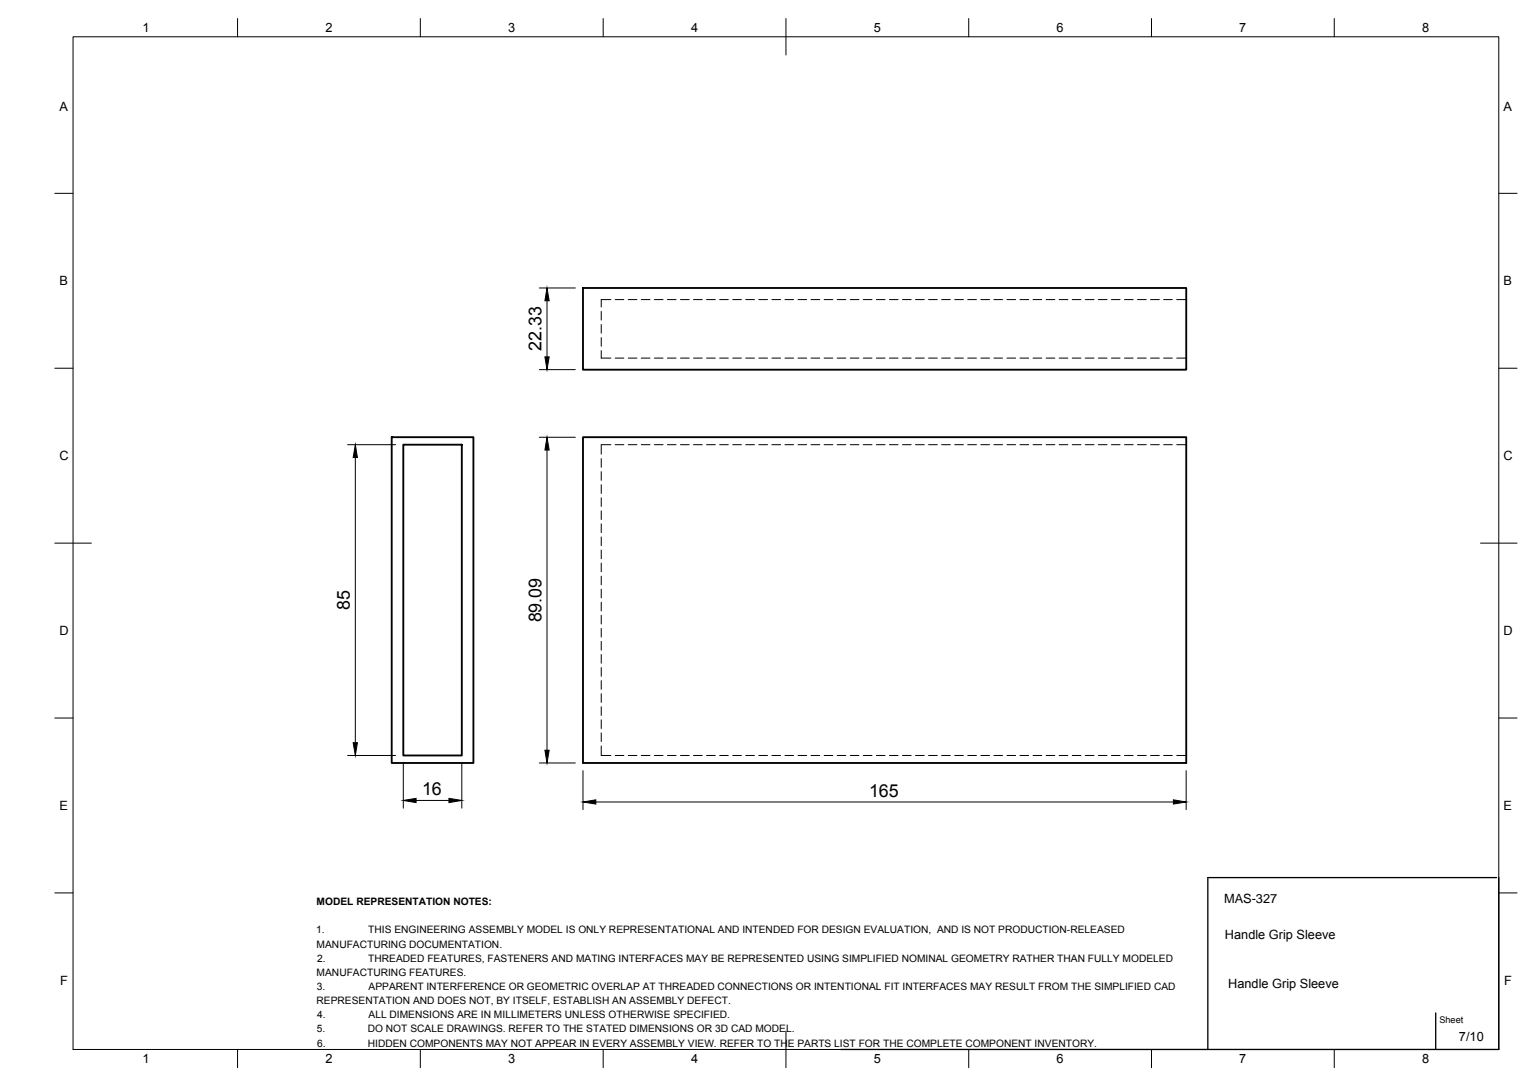
ISO-10303-21;
HEADER;
FILE_DESCRIPTION (('STEP AP214'),
    '1' );
FILE_NAME ('Handle Grip Sleeve.step',
    '2026-10-06T22:16:42',
    ( '' ),
    ( '' ),
    'SwSTEP 2.0',
    'SolidWorks 2025',
    '' );
FILE_SCHEMA (( 'AUTOMOTIVE_DESIGN' ));
ENDSEC;

DATA;
#37=ORIENTED_EDGE ( 'NONE', *, *, #161, .T. ) ;
#47=CARTESIAN_POINT ( 'NONE',  ( 2.004595370269653287, 635.3380690778678854, -0.8325491102011938205 ) ) ;
#122=CARTESIAN_POINT ( 'NONE',  ( -55.11860757350579831, 784.8075632535900468, -19.99999999999997868 ) ) ;
#123=ORIENTED_EDGE ( 'NONE', *, *, #17302, .F. ) ;
#161=EDGE_CURVE ( 'NONE', #6406, #8778, #2868, .T. ) ;
#223=ORIENTED_EDGE ( 'NONE', *, *, #18510, .T. ) ;
#234=PLANE ( 'NONE',  #15635 ) ;
#305=EDGE_CURVE ( 'NONE', #10554, #5083, #3643, .T. ) ;
#371=CARTESIAN_POINT ( 'NONE',  ( 0.08333186253070556937, 634.6318465664363657, -3.999999999999996447 ) ) ;
#441=DIRECTION ( 'NONE',  ( 0.000000000000000000, 0.000000000000000000, -1.000000000000000000 ) ) ;
#454=DIRECTION ( 'NONE',  ( 0.3450121214752279175, -0.9385982292947087080, 0.000000000000000000 ) ) ;
#567=CARTESIAN_POINT ( 'NONE',  ( -81.61981105773979550, 604.5992151483073940, -0.8325491102011938205 ) ) ;
#631=ORIENTED_EDGE ( 'NONE', *, *, #10728, .F. ) ;
#770=AXIS2_PLACEMENT_3D ( 'NONE', #10420, #3801, #12272 ) ;
#955=CARTESIAN_POINT ( 'NONE',  ( -134.9004869860375777, 755.4811543468929358, -19.99999999999996092 ) ) ;
#1022=CARTESIAN_POINT ( 'NONE',  ( -55.11860757350579831, 784.8075632535900468, -3.999999999999996447 ) ) ;
#1068=FACE_OUTER_BOUND ( 'NONE', #16645, .T. ) ;
#1109=ORIENTED_EDGE ( 'NONE', *, *, #17157, .T. ) ;
#1197=LINE ( 'NONE', #6263, #13695 ) ;
#1300=CARTESIAN_POINT ( 'NONE',  ( 0.08333186253067781379, 634.6318465664365931, -19.99999999999997868 ) ) ;
#1431=LINE ( 'NONE', #10574, #2685 ) ;
#1557=DIRECTION ( 'NONE',  ( -0.3450121214752279175, 0.9385982292947087080, 0.000000000000000000 ) ) ;
#1616=DIRECTION ( 'NONE',  ( 0.000000000000000000, 0.000000000000000000, -1.000000000000000000 ) ) ;
#1663=VECTOR ( 'NONE', #13216, 1000.000000000000114 ) ;
#1715=CARTESIAN_POINT ( 'NONE',  ( 0.08333186253067781379, 634.6318465664365931, -3.999999999999996447 ) ) ;
#1787=DIRECTION ( 'NONE',  ( 0.3450121214752279175, -0.9385982292947087080, -0.000000000000000000 ) ) ;
#1831=ORIENTED_EDGE ( 'NONE', *, *, #17120, .T. ) ;
#2049=ORIENTED_EDGE ( 'NONE', *, *, #6385, .T. ) ;
#2195=VECTOR ( 'NONE', #5994, 1000.000000000000000 ) ;
#2240=UNCERTAINTY_MEASURE_WITH_UNIT (LENGTH_MEASURE( 1.000000000000000082E-05 ), #9375, 'distance_accuracy_value', 'NONE');
#2256=ORIENTED_EDGE ( 'NONE', *, *, #305, .F. ) ;
#2403=CARTESIAN_POINT ( 'NONE',  ( 0.000000000000000000, 0.000000000000000000, 0.000000000000000000 ) ) ;
#2452=DIRECTION ( 'NONE',  ( 1.000000000000000000, 0.000000000000000000, -1.723963091245776585E-16 ) ) ;
#2568=LINE ( 'NONE', #2671, #12905 ) ;
#2635=FILL_AREA_STYLE ('',( #6156 ) ) ;
#2671=CARTESIAN_POINT ( 'NONE',  ( -138.5468111011521160, 759.4679229819337252, -0.8325491102011938205 ) ) ;
#2685=VECTOR ( 'NONE', #15626, 1000.000000000000000 ) ;
#2721=AXIS2_PLACEMENT_3D ( 'NONE', #1022, #14760, #2452 ) ;
#2868=LINE ( 'NONE', #18073, #21489 ) ;
#2903=ADVANCED_FACE ( 'NONE', ( #8379 ), #20176, .T. ) ;
#2927=VERTEX_POINT ( 'NONE', #11262 ) ;
#2952=VECTOR ( 'NONE', #1787, 1000.000000000000114 ) ;
#2972=AXIS2_PLACEMENT_3D ( 'NONE', #5225, #5530, #11012 ) ;
#3024=LINE ( 'NONE', #18003, #3512 ) ;
#3044=DIRECTION ( 'NONE',  ( -1.915514545828640705E-16, -7.041092946335507105E-17, -1.000000000000000000 ) ) ;
#3074=CARTESIAN_POINT ( 'NONE',  ( -81.61981105773979550, 604.5992151483073940, -23.16745088979876499 ) ) ;
#3090=ORIENTED_EDGE ( 'NONE', *, *, #18510, .F. ) ;
#3128=ORIENTED_EDGE ( 'NONE', *, *, #7265, .F. ) ;
#3197=LINE ( 'NONE', #6738, #17161 ) ;
#3211=FACE_OUTER_BOUND ( 'NONE', #21508, .T. ) ;
#3289=ORIENTED_EDGE ( 'NONE', *, *, #9467, .T. ) ;
#3512=VECTOR ( 'NONE', #12725, 1000.000000000000000 ) ;
#3514=ORIENTED_EDGE ( 'NONE', *, *, #12179, .F. ) ;
#3565=LINE ( 'NONE', #567, #6404 ) ;
#3643=LINE ( 'NONE', #5186, #7066 ) ;
#3693=FACE_OUTER_BOUND ( 'NONE', #13506, .T. ) ;
#3778=CARTESIAN_POINT ( 'NONE',  ( -55.11860757350579831, 784.8075632535900468, -3.999999999999996447 ) ) ;
#3801=DIRECTION ( 'NONE',  ( -0.9385982292947087080, -0.3450121214752279175, 0.000000000000000000 ) ) ;
#3806=DIRECTION ( 'NONE',  ( 0.9385982292947087080, 0.3450121214752278620, 0.000000000000000000 ) ) ;
#3809=VERTEX_POINT ( 'NONE', #21588 ) ;
#3912=LINE ( 'NONE', #4228, #8366 ) ;
#3957=CARTESIAN_POINT ( 'NONE',  ( -134.9004869860375777, 755.4811543468929358, -19.99999999999996092 ) ) ;
#3997=ORIENTED_EDGE ( 'NONE', *, *, #7265, .T. ) ;
#4161=COLOUR_RGB ( '', 0.08235294, 0.09019608, 0.10196078) ;
#4192=AXIS2_PLACEMENT_3D ( 'NONE', #955, #3044, #7699 ) ;
#4228=CARTESIAN_POINT ( 'NONE',  ( -79.69854755000110913, 605.3054376597395958, -19.99999999999996092 ) ) ;
#4444=VECTOR ( 'NONE', #17844, 1000.000000000000000 ) ;
#4545=VECTOR ( 'NONE', #21609, 1000.000000000000000 ) ;
#4608=FACE_OUTER_BOUND ( 'NONE', #15828, .T. ) ;
#4760=EDGE_LOOP ( 'NONE', ( #3128, #14818, #19148, #17206 ) ) ;
#4788=EDGE_CURVE ( 'NONE', #3809, #17748, #3912, .T. ) ;
#4797=PLANE ( 'NONE',  #8158 ) ;
#4869=MECHANICAL_DESIGN_GEOMETRIC_PRESENTATION_REPRESENTATION('',(#20026),#15063);
#5083=VERTEX_POINT ( 'NONE', #8870 ) ;
#5085=PLANE ( 'NONE',  #7827 ) ;
#5105=VERTEX_POINT ( 'NONE', #7431 ) ;
#5119=DIRECTION ( 'NONE',  ( 0.3450121214752279175, -0.9385982292947087080, 0.000000000000000000 ) ) ;
#5122=LINE ( 'NONE', #47, #8024 ) ;
#5186=CARTESIAN_POINT ( 'NONE',  ( -134.9004869860375777, 755.4811543468929358, -3.999999999999980904 ) ) ;
#5218=DIRECTION ( 'NONE',  ( 0.000000000000000000, 0.000000000000000000, 1.000000000000000000 ) ) ;
#5225=CARTESIAN_POINT ( 'NONE',  ( -81.61981105773979550, 604.5992151483073940, -0.8325491102011938205 ) ) ;
#5321=DIRECTION ( 'NONE',  ( 0.3450121214752279175, -0.9385982292947087080, -0.000000000000000000 ) ) ;
#5425=ORIENTED_EDGE ( 'NONE', *, *, #6726, .T. ) ;
#5501=ORIENTED_EDGE ( 'NONE', *, *, #8819, .T. ) ;
#5530=DIRECTION ( 'NONE',  ( 0.000000000000000000, -0.000000000000000000, 1.000000000000000000 ) ) ;
#5641=ORIENTED_EDGE ( 'NONE', *, *, #21598, .T. ) ;
#5994=DIRECTION ( 'NONE',  ( -0.9385982292947087080, -0.3450121214752279730, -0.000000000000000000 ) ) ;
#6156=FILL_AREA_STYLE_COLOUR ( '', #4161 ) ;
#6263=CARTESIAN_POINT ( 'NONE',  ( -79.69854755000110913, 605.3054376597395958, -3.999999999999980904 ) ) ;
#6385=EDGE_CURVE ( 'NONE', #12631, #21815, #15059, .T. ) ;
#6404=VECTOR ( 'NONE', #17203, 1000.000000000000000 ) ;
#6406=VERTEX_POINT ( 'NONE', #18480 ) ;
#6427=ORIENTED_EDGE ( 'NONE', *, *, #9863, .F. ) ;
#6497=CARTESIAN_POINT ( 'NONE',  ( 2.004595370269653287, 635.3380690778678854, -23.16745088979876499 ) ) ;
#6726=EDGE_CURVE ( 'NONE', #21815, #16287, #9432, .T. ) ;
#6738=CARTESIAN_POINT ( 'NONE',  ( -55.11860757350579831, 784.8075632535900468, -19.99999999999997868 ) ) ;
#6788=CARTESIAN_POINT ( 'NONE',  ( -262.4284940691236443, 713.9312056531381359, 0.000000000000000000 ) ) ;
#6799=ORIENTED_EDGE ( 'NONE', *, *, #4788, .F. ) ;
#6873=EDGE_LOOP ( 'NONE', ( #14795, #16577, #123, #12391 ) ) ;
#6878=ORIENTED_EDGE ( 'NONE', *, *, #21598, .F. ) ;
#6999=FACE_OUTER_BOUND ( 'NONE', #14526, .T. ) ;
#7021=AXIS2_PLACEMENT_3D ( 'NONE', #8149, #11327, #13209 ) ;
#7050=DIRECTION ( 'NONE',  ( 0.000000000000000000, 0.000000000000000000, 1.000000000000000000 ) ) ;
#7066=VECTOR ( 'NONE', #441, 1000.000000000000000 ) ;
#7076=ADVANCED_FACE ( 'NONE', ( #14914 ), #11944, .T. ) ;
#7121=ORIENTED_EDGE ( 'NONE', *, *, #20373, .F. ) ;
#7141=MANIFOLD_SOLID_BREP ( 'Cut-Extrude13', #16898 ) ;
#7265=EDGE_CURVE ( 'NONE', #16287, #5105, #18404, .T. ) ;
#7327=PLANE ( 'NONE',  #2721 ) ;
#7405=FACE_OUTER_BOUND ( 'NONE', #6873, .T. ) ;
#7431=CARTESIAN_POINT ( 'NONE',  ( -138.5468111011521160, 759.4679229819337252, -0.8325491102011938205 ) ) ;
#7446=ORIENTED_EDGE ( 'NONE', *, *, #12478, .F. ) ;
#7548=ORIENTED_EDGE ( 'NONE', *, *, #8548, .T. ) ;
#7699=DIRECTION ( 'NONE',  ( -1.000000000000000000, 0.000000000000000000, 1.915514545828640705E-16 ) ) ;
#7827=AXIS2_PLACEMENT_3D ( 'NONE', #122, #16647, #1557 ) ;
#7835=SURFACE_STYLE_USAGE ( .BOTH. , #19293 ) ;
#7863=CARTESIAN_POINT ( 'NONE',  ( -134.9004869860375777, 755.4811543468929358, -3.999999999999980904 ) ) ;
#7983=LINE ( 'NONE', #10072, #12722 ) ;
#7994=DIRECTION ( 'NONE',  ( 0.9385982292947087080, 0.3450121214752278620, -2.040824802394967678E-16 ) ) ;
#8024=VECTOR ( 'NONE', #18677, 1000.000000000000114 ) ;
#8051=DIRECTION ( 'NONE',  ( -0.9385982292947088190, -0.3450121214752275289, 0.000000000000000000 ) ) ;
#8149=CARTESIAN_POINT ( 'NONE',  ( 2.004595370269653287, 635.3380690778678854, -0.8325491102011938205 ) ) ;
#8158=AXIS2_PLACEMENT_3D ( 'NONE', #11518, #12276, #3806 ) ;
#8270=CARTESIAN_POINT ( 'NONE',  ( -138.5468111011521160, 759.4679229819337252, -0.8325491102011938205 ) ) ;
#8366=VECTOR ( 'NONE', #10639, 1000.000000000000000 ) ;
#8379=FACE_OUTER_BOUND ( 'NONE', #4760, .T. ) ;
#8434=CARTESIAN_POINT ( 'NONE',  ( -81.61981105773979550, 604.5992151483073940, -23.16745088979876499 ) ) ;
#8494=DIRECTION ( 'NONE',  ( 0.3450121214752279175, -0.9385982292947087080, -0.000000000000000000 ) ) ;
#8540=ORIENTED_EDGE ( 'NONE', *, *, #6726, .F. ) ;
#8548=EDGE_CURVE ( 'NONE', #13406, #19098, #13505, .T. ) ;
#8778=VERTEX_POINT ( 'NONE', #16123 ) ;
#8819=EDGE_CURVE ( 'NONE', #5105, #12631, #2568, .T. ) ;
#8870=CARTESIAN_POINT ( 'NONE',  ( -134.9004869860375777, 755.4811543468929358, -19.99999999999996092 ) ) ;
#9128=ORIENTED_EDGE ( 'NONE', *, *, #9740, .T. ) ;
#9147=VECTOR ( 'NONE', #13213, 1000.000000000000114 ) ;
#9349=SHAPE_REPRESENTATION_RELATIONSHIP ( 'NONE' , 'NONE' ,  #21416, #10590 ) ;
#9372=VECTOR ( 'NONE', #13820, 1000.000000000000000 ) ;
#9375=( LENGTH_UNIT ( ) NAMED_UNIT ( * ) SI_UNIT ( .MILLI., .METRE. ) );
#9432=LINE ( 'NONE', #9541, #2195 ) ;
#9467=EDGE_CURVE ( 'NONE', #8778, #10077, #12458, .T. ) ;
#9541=CARTESIAN_POINT ( 'NONE',  ( -138.5468111011521160, 759.4679229819337252, -23.16745088979876499 ) ) ;
#9654=PRODUCT_CONTEXT ( 'NONE', #21405, 'mechanical' ) ;
#9740=EDGE_CURVE ( 'NONE', #10077, #2927, #1431, .T. ) ;
#9863=EDGE_CURVE ( 'NONE', #5083, #3809, #13758, .T. ) ;
#9969=ORIENTED_EDGE ( 'NONE', *, *, #11352, .F. ) ;
#10033=CARTESIAN_POINT ( 'NONE',  ( -79.69854755000110913, 605.3054376597395958, -3.999999999999980904 ) ) ;
#10072=CARTESIAN_POINT ( 'NONE',  ( -55.11860757350579831, 784.8075632535900468, -3.999999999999996447 ) ) ;
#10077=VERTEX_POINT ( 'NONE', #19269 ) ;
#10162=ORIENTED_EDGE ( 'NONE', *, *, #12179, .T. ) ;
#10297=FACE_OUTER_BOUND ( 'NONE', #18443, .T. ) ;
#10420=CARTESIAN_POINT ( 'NONE',  ( -134.9004869860375777, 755.4811543468929358, -3.999999999999980904 ) ) ;
#10435=AXIS2_PLACEMENT_3D ( 'NONE', #11779, #8051, #15088 ) ;
#10507=CARTESIAN_POINT ( 'NONE',  ( -55.11860757350579831, 784.8075632535900468, -19.99999999999997868 ) ) ;
#10554=VERTEX_POINT ( 'NONE', #21663 ) ;
#10574=CARTESIAN_POINT ( 'NONE',  ( -81.61981105773979550, 604.5992151483073940, -23.16745088979876499 ) ) ;
#10590=ADVANCED_BREP_SHAPE_REPRESENTATION ( '', ( #7141, #12657 ), #17239 ) ;
#10639=DIRECTION ( 'NONE',  ( 0.9385982292947087080, 0.3450121214752278620, -2.040824802394967678E-16 ) ) ;
#10728=EDGE_CURVE ( 'NONE', #5083, #21052, #19666, .T. ) ;
#11012=DIRECTION ( 'NONE',  ( 1.000000000000000000, 0.000000000000000000, -0.000000000000000000 ) ) ;
#11071=PRODUCT_DEFINITION ( 'UNKNOWN', '', #13384, #13252 ) ;
#11090=CARTESIAN_POINT ( 'NONE',  ( -55.11860757350579831, 784.8075632535900468, -19.99999999999997868 ) ) ;
#11140=VECTOR ( 'NONE', #8494, 1000.000000000000114 ) ;
#11199=CARTESIAN_POINT ( 'NONE',  ( -81.61981105773979550, 604.5992151483073940, -0.8325491102011938205 ) ) ;
#11229=PRESENTATION_STYLE_ASSIGNMENT (( #7835 ) ) ;
#11262=CARTESIAN_POINT ( 'NONE',  ( -81.61981105773979550, 604.5992151483073940, -23.16745088979876499 ) ) ;
#11288=SHAPE_DEFINITION_REPRESENTATION ( #16260, #21416 ) ;
#11309=( NAMED_UNIT ( * ) PLANE_ANGLE_UNIT ( ) SI_UNIT ( $, .RADIAN. ) );
#11327=DIRECTION ( 'NONE',  ( 0.9385982292947088190, 0.3450121214752275289, 0.000000000000000000 ) ) ;
#11352=EDGE_CURVE ( 'NONE', #10077, #21815, #21495, .T. ) ;
#11518=CARTESIAN_POINT ( 'NONE',  ( -260.7034334617478066, 709.2382145066653720, 0.000000000000000000 ) ) ;
#11543=APPLICATION_CONTEXT ( 'automotive_design' ) ;
#11566=CARTESIAN_POINT ( 'NONE',  ( -54.92240467314265828, 790.2067769114943303, -0.8325491102011938205 ) ) ;
#11714=ORIENTED_EDGE ( 'NONE', *, *, #6385, .F. ) ;
#11779=CARTESIAN_POINT ( 'NONE',  ( -81.61981105773979550, 604.5992151483073940, -0.8325491102011938205 ) ) ;
#11944=PLANE ( 'NONE',  #14365 ) ;
#12020=DIRECTION ( 'NONE',  ( 0.9385982292947087080, 0.3450121214752279175, 0.000000000000000000 ) ) ;
#12179=EDGE_CURVE ( 'NONE', #8778, #12631, #5122, .T. ) ;
#12250=EDGE_LOOP ( 'NONE', ( #1831, #20399, #14015, #15592 ) ) ;
#12272=DIRECTION ( 'NONE',  ( 0.3450121214752279175, -0.9385982292947087080, 0.000000000000000000 ) ) ;
#12276=DIRECTION ( 'NONE',  ( 0.3450121214752278620, -0.9385982292947087080, 0.000000000000000000 ) ) ;
#12333=ORIENTED_EDGE ( 'NONE', *, *, #21480, .T. ) ;
#12385=VECTOR ( 'NONE', #1616, 1000.000000000000000 ) ;
#12391=ORIENTED_EDGE ( 'NONE', *, *, #9740, .F. ) ;
#12425=ADVANCED_FACE ( 'NONE', ( #21502 ), #7327, .F. ) ;
#12457=CARTESIAN_POINT ( 'NONE',  ( -205.5014940257113665, 559.0624978195118047, 0.000000000000000000 ) ) ;
#12458=LINE ( 'NONE', #14433, #4444 ) ;
#12478=EDGE_CURVE ( 'NONE', #21052, #17748, #3197, .T. ) ;
#12523=ORIENTED_EDGE ( 'NONE', *, *, #8819, .F. ) ;
#12631=VERTEX_POINT ( 'NONE', #11566 ) ;
#12639=EDGE_LOOP ( 'NONE', ( #8540, #9969, #9128, #12333 ) ) ;
#12657=AXIS2_PLACEMENT_3D ( 'NONE', #2403, #7050, #17169 ) ;
#12722=VECTOR ( 'NONE', #16781, 1000.000000000000000 ) ;
#12725=DIRECTION ( 'NONE',  ( 0.000000000000000000, 0.000000000000000000, 1.000000000000000000 ) ) ;
#12905=VECTOR ( 'NONE', #17444, 1000.000000000000000 ) ;
#12975=( LENGTH_UNIT ( ) NAMED_UNIT ( * ) SI_UNIT ( .MILLI., .METRE. ) );
#13092=VECTOR ( 'NONE', #5321, 1000.000000000000114 ) ;
#13144=ORIENTED_EDGE ( 'NONE', *, *, #20373, .T. ) ;
#13183=LINE ( 'NONE', #11199, #16866 ) ;
#13209=DIRECTION ( 'NONE',  ( -0.3450121214752275289, 0.9385982292947088190, 0.000000000000000000 ) ) ;
#13213=DIRECTION ( 'NONE',  ( -0.3450121214752274734, 0.9385982292947088190, 0.000000000000000000 ) ) ;
#13216=DIRECTION ( 'NONE',  ( -0.3450121214752274734, 0.9385982292947088190, 0.000000000000000000 ) ) ;
#13252=PRODUCT_DEFINITION_CONTEXT ( 'detailed design', #11543, 'design' ) ;
#13279=DIRECTION ( 'NONE',  ( 0.000000000000000000, 0.000000000000000000, -1.000000000000000000 ) ) ;
#13384=PRODUCT_DEFINITION_FORMATION_WITH_SPECIFIED_SOURCE ( 'ANY', '', #21567, .NOT_KNOWN. ) ;
#13406=VERTEX_POINT ( 'NONE', #371 ) ;
#13505=LINE ( 'NONE', #1715, #9372 ) ;
#13506=EDGE_LOOP ( 'NONE', ( #13144, #6427, #2256, #223 ) ) ;
#13695=VECTOR ( 'NONE', #18050, 1000.000000000000000 ) ;
#13703=DIRECTION ( 'NONE',  ( 0.9385982292947087080, 0.3450121214752279175, 0.000000000000000000 ) ) ;
#13713=CARTESIAN_POINT ( 'NONE',  ( -138.5468111011521160, 759.4679229819337252, -23.16745088979876499 ) ) ;
#13758=LINE ( 'NONE', #3957, #11140 ) ;
#13820=DIRECTION ( 'NONE',  ( -0.9385982292947087080, -0.3450121214752278620, 1.836742322155470738E-16 ) ) ;
#13835=CARTESIAN_POINT ( 'NONE',  ( -54.92240467314265828, 790.2067769114943303, -0.8325491102011938205 ) ) ;
#13966=VECTOR ( 'NONE', #7994, 1000.000000000000000 ) ;
#14015=ORIENTED_EDGE ( 'NONE', *, *, #305, .T. ) ;
#14322=( NAMED_UNIT ( * ) PLANE_ANGLE_UNIT ( ) SI_UNIT ( $, .RADIAN. ) );
#14355=ORIENTED_EDGE ( 'NONE', *, *, #12478, .T. ) ;
#14365=AXIS2_PLACEMENT_3D ( 'NONE', #8434, #13279, #18345 ) ;
#14433=CARTESIAN_POINT ( 'NONE',  ( 2.004595370269653287, 635.3380690778678854, -0.8325491102011938205 ) ) ;
#14526=EDGE_LOOP ( 'NONE', ( #2049, #5425, #3997, #5501 ) ) ;
#14664=ADVANCED_FACE ( 'NONE', ( #3211 ), #5085, .F. ) ;
#14760=DIRECTION ( 'NONE',  ( 1.723963091245776585E-16, 6.336983651701956765E-17, 1.000000000000000000 ) ) ;
#14795=ORIENTED_EDGE ( 'NONE', *, *, #9467, .F. ) ;
#14818=ORIENTED_EDGE ( 'NONE', *, *, #21480, .F. ) ;
#14841=PLANE ( 'NONE',  #770 ) ;
#14901=ORIENTED_EDGE ( 'NONE', *, *, #8548, .F. ) ;
#14914=FACE_OUTER_BOUND ( 'NONE', #12639, .T. ) ;
#15047=FACE_OUTER_BOUND ( 'NONE', #12250, .T. ) ;
#15059=LINE ( 'NONE', #13835, #12385 ) ;
#15063=( GEOMETRIC_REPRESENTATION_CONTEXT ( 3 ) GLOBAL_UNCERTAINTY_ASSIGNED_CONTEXT ( ( #2240 ) ) GLOBAL_UNIT_ASSIGNED_CONTEXT ( ( #9375, #14322, #17841 ) ) REPRESENTATION_CONTEXT ( 'NONE', 'WORKASPACE' ) );
#15088=DIRECTION ( 'NONE',  ( 0.3450121214752275289, -0.9385982292947088190, 0.000000000000000000 ) ) ;
#15246=LINE ( 'NONE', #18662, #13092 ) ;
#15261=UNCERTAINTY_MEASURE_WITH_UNIT (LENGTH_MEASURE( 1.000000000000000082E-05 ), #12975, 'distance_accuracy_value', 'NONE');
#15333=EDGE_LOOP ( 'NONE', ( #7548, #3090, #16968, #1109 ) ) ;
#15342=FACE_BOUND ( 'NONE', #20311, .T. ) ;
#15440=ORIENTED_EDGE ( 'NONE', *, *, #17157, .F. ) ;
#15592=ORIENTED_EDGE ( 'NONE', *, *, #10728, .T. ) ;
#15626=DIRECTION ( 'NONE',  ( -0.9385982292947087080, -0.3450121214752279730, -0.000000000000000000 ) ) ;
#15635=AXIS2_PLACEMENT_3D ( 'NONE', #12457, #454, #12020 ) ;
#15828=EDGE_LOOP ( 'NONE', ( #11714, #3514, #3289, #18695 ) ) ;
#16043=PLANE ( 'NONE',  #4192 ) ;
#16056=ADVANCED_FACE ( 'NONE', ( #3693 ), #14841, .F. ) ;
#16123=CARTESIAN_POINT ( 'NONE',  ( 2.004595370269653287, 635.3380690778678854, -0.8325491102011938205 ) ) ;
#16189=SURFACE_STYLE_FILL_AREA ( #2635 ) ;
#16218=LINE ( 'NONE', #7863, #2952 ) ;
#16260=PRODUCT_DEFINITION_SHAPE ( 'NONE', 'NONE',  #11071 ) ;
#16287=VERTEX_POINT ( 'NONE', #13713 ) ;
#16397=ADVANCED_FACE ( 'NONE', ( #15047 ), #4797, .T. ) ;
#16577=ORIENTED_EDGE ( 'NONE', *, *, #161, .F. ) ;
#16645=EDGE_LOOP ( 'NONE', ( #19149, #7446, #631, #18609 ) ) ;
#16647=DIRECTION ( 'NONE',  ( 0.9385982292947087080, 0.3450121214752279175, -0.000000000000000000 ) ) ;
#16781=DIRECTION ( 'NONE',  ( -0.9385982292947087080, -0.3450121214752278620, 1.836742322155470738E-16 ) ) ;
#16847=DIRECTION ( 'NONE',  ( 0.3450121214752279175, -0.9385982292947087080, -0.000000000000000000 ) ) ;
#16866=VECTOR ( 'NONE', #19805, 1000.000000000000114 ) ;
#16898=CLOSED_SHELL ( 'NONE', ( #20263, #19897, #2903, #7076, #18687, #18101, #14664, #21046, #16056, #12425, #16397 ) ) ;
#16967=EDGE_CURVE ( 'NONE', #17262, #10554, #7983, .T. ) ;
#16968=ORIENTED_EDGE ( 'NONE', *, *, #16967, .F. ) ;
#17006=PLANE ( 'NONE',  #21200 ) ;
#17120=EDGE_CURVE ( 'NONE', #21052, #17262, #17316, .T. ) ;
#17157=EDGE_CURVE ( 'NONE', #17262, #13406, #15246, .T. ) ;
#17161=VECTOR ( 'NONE', #16847, 1000.000000000000114 ) ;
#17169=DIRECTION ( 'NONE',  ( 1.000000000000000000, 0.000000000000000000, 0.000000000000000000 ) ) ;
#17203=DIRECTION ( 'NONE',  ( -0.000000000000000000, -0.000000000000000000, 1.000000000000000000 ) ) ;
#17206=ORIENTED_EDGE ( 'NONE', *, *, #20919, .T. ) ;
#17239=( GEOMETRIC_REPRESENTATION_CONTEXT ( 3 ) GLOBAL_UNCERTAINTY_ASSIGNED_CONTEXT ( ( #15261 ) ) GLOBAL_UNIT_ASSIGNED_CONTEXT ( ( #12975, #11309, #19477 ) ) REPRESENTATION_CONTEXT ( 'NONE', 'WORKASPACE' ) );
#17262=VERTEX_POINT ( 'NONE', #3778 ) ;
#17302=EDGE_CURVE ( 'NONE', #2927, #6406, #3565, .T. ) ;
#17316=LINE ( 'NONE', #10507, #19411 ) ;
#17444=DIRECTION ( 'NONE',  ( 0.9385982292947087080, 0.3450121214752279730, 0.000000000000000000 ) ) ;
#17748=VERTEX_POINT ( 'NONE', #1300 ) ;
#17841=( NAMED_UNIT ( * ) SI_UNIT ( $, .STERADIAN. ) SOLID_ANGLE_UNIT ( ) );
#17844=DIRECTION ( 'NONE',  ( 0.000000000000000000, 0.000000000000000000, -1.000000000000000000 ) ) ;
#17938=PLANE ( 'NONE',  #7021 ) ;
#18003=CARTESIAN_POINT ( 'NONE',  ( 0.08333186253067781379, 634.6318465664365931, -19.99999999999997868 ) ) ;
#18050=DIRECTION ( 'NONE',  ( 0.000000000000000000, 0.000000000000000000, -1.000000000000000000 ) ) ;
#18073=CARTESIAN_POINT ( 'NONE',  ( -81.61981105773979550, 604.5992151483073940, -0.8325491102011938205 ) ) ;
#18101=ADVANCED_FACE ( 'NONE', ( #6999 ), #17006, .F. ) ;
#18166=LINE ( 'NONE', #3074, #9147 ) ;
#18187=DIRECTION ( 'NONE',  ( 0.9385982292947087080, 0.3450121214752279730, 0.000000000000000000 ) ) ;
#18345=DIRECTION ( 'NONE',  ( -1.000000000000000000, 0.000000000000000000, -0.000000000000000000 ) ) ;
#18404=LINE ( 'NONE', #8270, #4545 ) ;
#18443=EDGE_LOOP ( 'NONE', ( #12523, #21072, #37, #10162 ) ) ;
#18480=CARTESIAN_POINT ( 'NONE',  ( -81.61981105773979550, 604.5992151483073940, -0.8325491102011938205 ) ) ;
#18510=EDGE_CURVE ( 'NONE', #10554, #19098, #16218, .T. ) ;
#18609=ORIENTED_EDGE ( 'NONE', *, *, #9863, .T. ) ;
#18662=CARTESIAN_POINT ( 'NONE',  ( -55.11860757350579831, 784.8075632535900468, -3.999999999999996447 ) ) ;
#18677=DIRECTION ( 'NONE',  ( -0.3450121214752274734, 0.9385982292947088190, 0.000000000000000000 ) ) ;
#18687=ADVANCED_FACE ( 'NONE', ( #15342, #7405 ), #234, .T. ) ;
#18695=ORIENTED_EDGE ( 'NONE', *, *, #11352, .T. ) ;
#18833=CARTESIAN_POINT ( 'NONE',  ( -54.92240467314265828, 790.2067769114943303, -23.16745088979876499 ) ) ;
#18878=PLANE ( 'NONE',  #2972 ) ;
#19098=VERTEX_POINT ( 'NONE', #10033 ) ;
#19148=ORIENTED_EDGE ( 'NONE', *, *, #17302, .T. ) ;
#19149=ORIENTED_EDGE ( 'NONE', *, *, #4788, .T. ) ;
#19269=CARTESIAN_POINT ( 'NONE',  ( 2.004595370269653287, 635.3380690778678854, -23.16745088979876499 ) ) ;
#19293=SURFACE_SIDE_STYLE ('',( #16189 ) ) ;
#19411=VECTOR ( 'NONE', #5218, 1000.000000000000000 ) ;
#19477=( NAMED_UNIT ( * ) SI_UNIT ( $, .STERADIAN. ) SOLID_ANGLE_UNIT ( ) );
#19666=LINE ( 'NONE', #21436, #13966 ) ;
#19761=ORIENTED_EDGE ( 'NONE', *, *, #17120, .F. ) ;
#19805=DIRECTION ( 'NONE',  ( -0.3450121214752274734, 0.9385982292947088190, 0.000000000000000000 ) ) ;
#19897=ADVANCED_FACE ( 'NONE', ( #10297 ), #18878, .T. ) ;
#20026=STYLED_ITEM ( 'NONE', ( #11229 ), #7141 ) ;
#20176=PLANE ( 'NONE',  #10435 ) ;
#20263=ADVANCED_FACE ( 'NONE', ( #4608 ), #17938, .T. ) ;
#20311=EDGE_LOOP ( 'NONE', ( #6878, #6799, #7121, #14901 ) ) ;
#20373=EDGE_CURVE ( 'NONE', #19098, #3809, #1197, .T. ) ;
#20399=ORIENTED_EDGE ( 'NONE', *, *, #16967, .T. ) ;
#20919=EDGE_CURVE ( 'NONE', #6406, #5105, #13183, .T. ) ;
#21046=ADVANCED_FACE ( 'NONE', ( #1068 ), #16043, .F. ) ;
#21052=VERTEX_POINT ( 'NONE', #11090 ) ;
#21072=ORIENTED_EDGE ( 'NONE', *, *, #20919, .F. ) ;
#21200=AXIS2_PLACEMENT_3D ( 'NONE', #6788, #5119, #13703 ) ;
#21405=APPLICATION_CONTEXT ( 'automotive_design' ) ;
#21416=SHAPE_REPRESENTATION ( 'Handle Grip Sleeve', ( #12657 ), #17239 ) ;
#21436=CARTESIAN_POINT ( 'NONE',  ( -134.9004869860375777, 755.4811543468929358, -19.99999999999996092 ) ) ;
#21480=EDGE_CURVE ( 'NONE', #2927, #16287, #18166, .T. ) ;
#21489=VECTOR ( 'NONE', #18187, 1000.000000000000000 ) ;
#21495=LINE ( 'NONE', #6497, #1663 ) ;
#21502=FACE_OUTER_BOUND ( 'NONE', #15333, .T. ) ;
#21508=EDGE_LOOP ( 'NONE', ( #5641, #15440, #19761, #14355 ) ) ;
#21567=PRODUCT ( 'Handle Grip Sleeve', 'Handle Grip Sleeve', '', ( #9654 ) ) ;
#21588=CARTESIAN_POINT ( 'NONE',  ( -79.69854755000110913, 605.3054376597395958, -19.99999999999996092 ) ) ;
#21598=EDGE_CURVE ( 'NONE', #17748, #13406, #3024, .T. ) ;
#21609=DIRECTION ( 'NONE',  ( -0.000000000000000000, -0.000000000000000000, 1.000000000000000000 ) ) ;
#21663=CARTESIAN_POINT ( 'NONE',  ( -134.9004869860375777, 755.4811543468929358, -3.999999999999980904 ) ) ;
#21815=VERTEX_POINT ( 'NONE', #18833 ) ;
ENDSEC;
END-ISO-10303-21;
